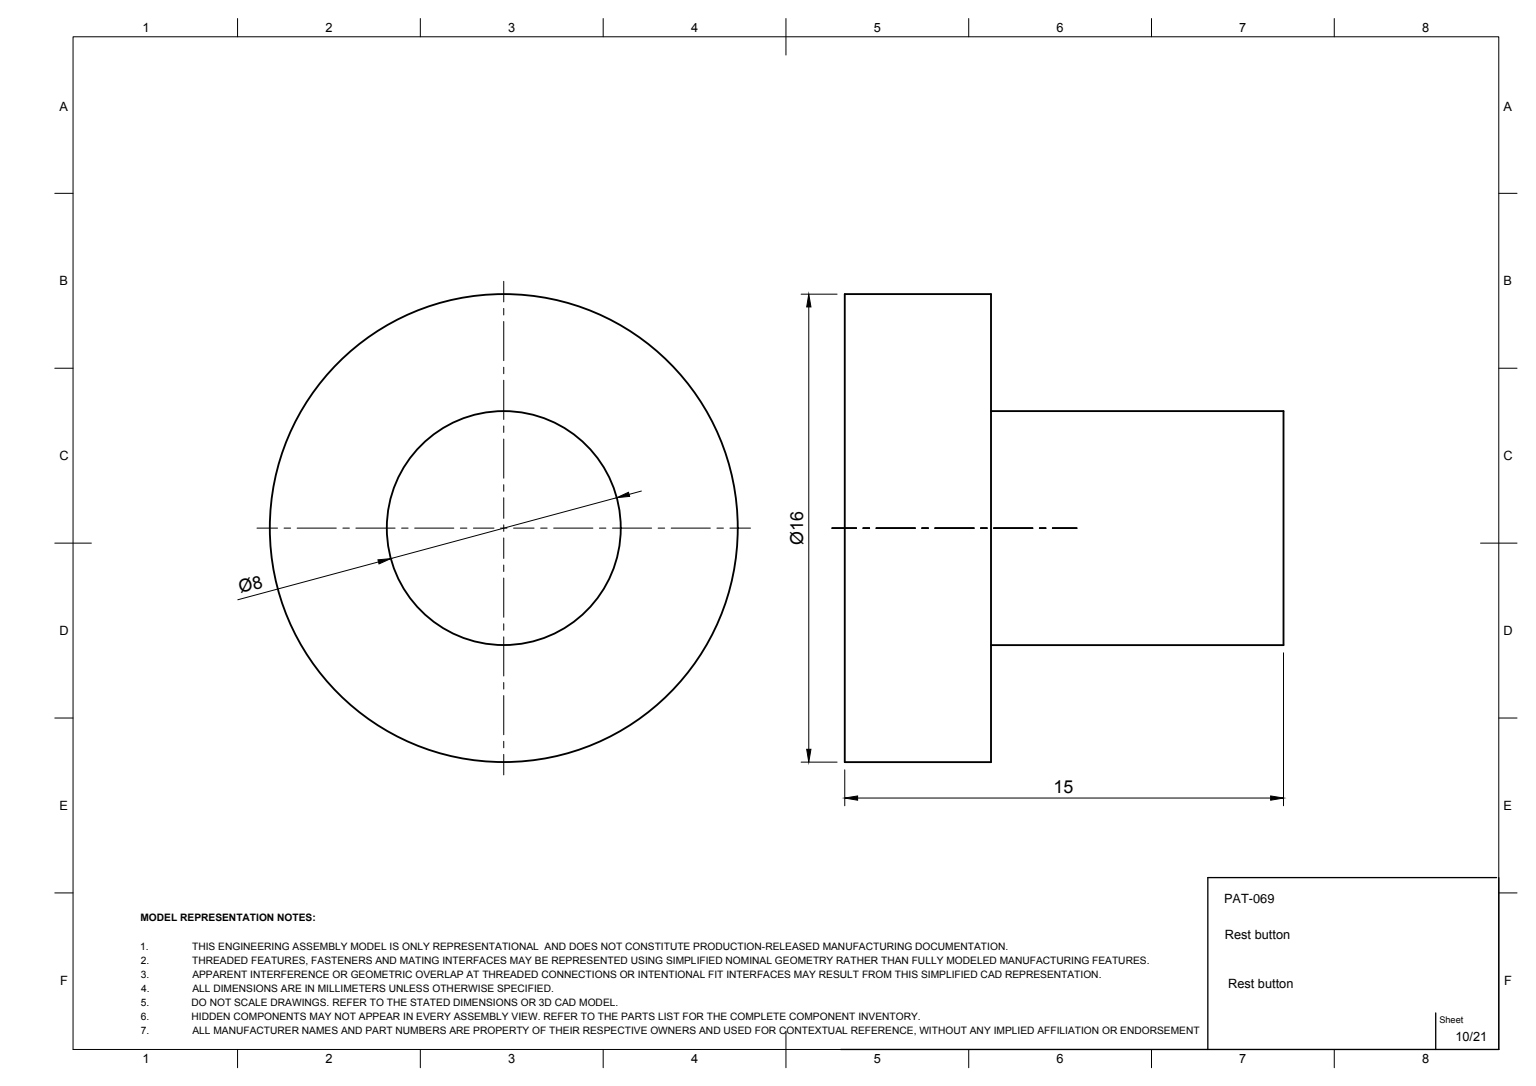
ISO-10303-21;
HEADER;
/* Generated by software containing ST-Developer
 * from STEP Tools, Inc. (www.steptools.com) 
 */

FILE_DESCRIPTION(
/* description */ ('Located fixture plate with toggle clamp'),
/* implementation_level */ '2;1');

FILE_NAME(
/* name */ 'Rest button.step',
/* time_stamp */ '2026-10-27T21:36:12-07:00',
/* author */ (''),
/* organization */ (''),
/* preprocessor_version */ 'ST-DEVELOPER v20.2',
/* originating_system */ 'Autodesk Translation Framework v15.17.0.0',
/* authorisation */ '');

FILE_SCHEMA (('AUTOMOTIVE_DESIGN { 1 0 10303 214 3 1 1 }'));
ENDSEC;

DATA;
#10=MECHANICAL_DESIGN_GEOMETRIC_PRESENTATION_REPRESENTATION('',(#329),#9285);
#281=SHAPE_REPRESENTATION_RELATIONSHIP('SRR','None',#9404,#305);
#305=ADVANCED_BREP_SHAPE_REPRESENTATION('',(#352),#9266);
#329=STYLED_ITEM('',(#9626),#352);
#352=MANIFOLD_SOLID_BREP('Body1',#5178);
#451=FACE_BOUND('',#1200,.T.);
#574=PLANE('',#5722);
#575=PLANE('',#5726);
#576=PLANE('',#5727);
#816=FACE_OUTER_BOUND('',#1196,.T.);
#817=FACE_OUTER_BOUND('',#1197,.T.);
#818=FACE_OUTER_BOUND('',#1198,.T.);
#819=FACE_OUTER_BOUND('',#1199,.T.);
#820=FACE_OUTER_BOUND('',#1201,.T.);
#1196=EDGE_LOOP('',(#4176,#4177,#4178,#4179));
#1197=EDGE_LOOP('',(#4180));
#1198=EDGE_LOOP('',(#4181,#4182,#4183,#4184));
#1199=EDGE_LOOP('',(#4185));
#1200=EDGE_LOOP('',(#4186));
#1201=EDGE_LOOP('',(#4187));
#1487=CIRCLE('',#5720,0.4);
#1488=CIRCLE('',#5721,0.4);
#1489=CIRCLE('',#5724,0.8);
#1490=CIRCLE('',#5725,0.8);
#1805=LINE('',#8343,#2215);
#1806=LINE('',#8350,#2216);
#2215=VECTOR('',#6773,0.4);
#2216=VECTOR('',#6782,0.8);
#2629=VERTEX_POINT('',#8340);
#2630=VERTEX_POINT('',#8342);
#2631=VERTEX_POINT('',#8347);
#2632=VERTEX_POINT('',#8349);
#3176=EDGE_CURVE('',#2629,#2629,#1487,.T.);
#3177=EDGE_CURVE('',#2629,#2630,#1805,.T.);
#3178=EDGE_CURVE('',#2630,#2630,#1488,.T.);
#3179=EDGE_CURVE('',#2631,#2631,#1489,.T.);
#3180=EDGE_CURVE('',#2631,#2632,#1806,.T.);
#3181=EDGE_CURVE('',#2632,#2632,#1490,.T.);
#4176=ORIENTED_EDGE('',*,*,#3176,.F.);
#4177=ORIENTED_EDGE('',*,*,#3177,.T.);
#4178=ORIENTED_EDGE('',*,*,#3178,.F.);
#4179=ORIENTED_EDGE('',*,*,#3177,.F.);
#4180=ORIENTED_EDGE('',*,*,#3176,.T.);
#4181=ORIENTED_EDGE('',*,*,#3179,.F.);
#4182=ORIENTED_EDGE('',*,*,#3180,.T.);
#4183=ORIENTED_EDGE('',*,*,#3181,.T.);
#4184=ORIENTED_EDGE('',*,*,#3180,.F.);
#4185=ORIENTED_EDGE('',*,*,#3179,.T.);
#4186=ORIENTED_EDGE('',*,*,#3178,.T.);
#4187=ORIENTED_EDGE('',*,*,#3181,.F.);
#4839=CYLINDRICAL_SURFACE('',#5719,0.4);
#4840=CYLINDRICAL_SURFACE('',#5723,0.8);
#5017=ADVANCED_FACE('',(#816),#4839,.T.);
#5018=ADVANCED_FACE('',(#817),#574,.T.);
#5019=ADVANCED_FACE('',(#818),#4840,.T.);
#5020=ADVANCED_FACE('',(#819,#451),#575,.T.);
#5021=ADVANCED_FACE('',(#820),#576,.F.);
#5178=CLOSED_SHELL('',(#5017,#5018,#5019,#5020,#5021));
#5718=AXIS2_PLACEMENT_3D('',#8338,#6767,#6768);
#5719=AXIS2_PLACEMENT_3D('',#8339,#6769,#6770);
#5720=AXIS2_PLACEMENT_3D('',#8341,#6771,#6772);
#5721=AXIS2_PLACEMENT_3D('',#8344,#6774,#6775);
#5722=AXIS2_PLACEMENT_3D('',#8345,#6776,#6777);
#5723=AXIS2_PLACEMENT_3D('',#8346,#6778,#6779);
#5724=AXIS2_PLACEMENT_3D('',#8348,#6780,#6781);
#5725=AXIS2_PLACEMENT_3D('',#8351,#6783,#6784);
#5726=AXIS2_PLACEMENT_3D('',#8352,#6785,#6786);
#5727=AXIS2_PLACEMENT_3D('',#8353,#6787,#6788);
#6767=DIRECTION('axis',(0.,0.,1.));
#6768=DIRECTION('refdir',(1.,0.,0.));
#6769=DIRECTION('center_axis',(1.,0.,0.));
#6770=DIRECTION('ref_axis',(0.,0.,-1.));
#6771=DIRECTION('center_axis',(1.,0.,0.));
#6772=DIRECTION('ref_axis',(0.,0.,-1.));
#6773=DIRECTION('',(-1.,0.,0.));
#6774=DIRECTION('center_axis',(-1.,0.,0.));
#6775=DIRECTION('ref_axis',(0.,0.,-1.));
#6776=DIRECTION('center_axis',(1.,0.,0.));
#6777=DIRECTION('ref_axis',(0.,0.,-1.));
#6778=DIRECTION('center_axis',(1.,0.,0.));
#6779=DIRECTION('ref_axis',(0.,0.,-1.));
#6780=DIRECTION('center_axis',(1.,0.,0.));
#6781=DIRECTION('ref_axis',(0.,0.,-1.));
#6782=DIRECTION('',(-1.,0.,0.));
#6783=DIRECTION('center_axis',(1.,0.,0.));
#6784=DIRECTION('ref_axis',(0.,0.,-1.));
#6785=DIRECTION('center_axis',(1.,0.,0.));
#6786=DIRECTION('ref_axis',(0.,0.,-1.));
#6787=DIRECTION('center_axis',(1.,0.,0.));
#6788=DIRECTION('ref_axis',(0.,0.,-1.));
#8338=CARTESIAN_POINT('',(0.,0.,0.));
#8339=CARTESIAN_POINT('Origin',(18.8,-2.5,2.));
#8340=CARTESIAN_POINT('',(19.8,-2.5,2.4));
#8341=CARTESIAN_POINT('Origin',(19.8,-2.5,2.));
#8342=CARTESIAN_POINT('',(18.8,-2.5,2.4));
#8343=CARTESIAN_POINT('',(18.8,-2.5,2.4));
#8344=CARTESIAN_POINT('Origin',(18.8,-2.5,2.));
#8345=CARTESIAN_POINT('Origin',(19.8,-2.5,2.));
#8346=CARTESIAN_POINT('Origin',(18.3,-2.5,2.));
#8347=CARTESIAN_POINT('',(18.8,-2.5,2.8));
#8348=CARTESIAN_POINT('Origin',(18.8,-2.5,2.));
#8349=CARTESIAN_POINT('',(18.3,-2.5,2.8));
#8350=CARTESIAN_POINT('',(18.3,-2.5,2.8));
#8351=CARTESIAN_POINT('Origin',(18.3,-2.5,2.));
#8352=CARTESIAN_POINT('Origin',(18.8,-2.5,2.));
#8353=CARTESIAN_POINT('Origin',(18.3,-2.5,2.));
#9236=UNCERTAINTY_MEASURE_WITH_UNIT(LENGTH_MEASURE(0.001),#9286,
'DISTANCE_ACCURACY_VALUE',
'Maximum model space distance between geometric entities at asserted c
onnectivities');
#9255=UNCERTAINTY_MEASURE_WITH_UNIT(LENGTH_MEASURE(0.001),#9286,
'DISTANCE_ACCURACY_VALUE',
'Maximum model space distance between geometric entities at asserted c
onnectivities');
#9266=(
GEOMETRIC_REPRESENTATION_CONTEXT(3)
GLOBAL_UNCERTAINTY_ASSIGNED_CONTEXT((#9236))
GLOBAL_UNIT_ASSIGNED_CONTEXT((#9286,#9288,#9289))
REPRESENTATION_CONTEXT('','3D')
);
#9285=(
GEOMETRIC_REPRESENTATION_CONTEXT(3)
GLOBAL_UNCERTAINTY_ASSIGNED_CONTEXT((#9255))
GLOBAL_UNIT_ASSIGNED_CONTEXT((#9286,#9288,#9289))
REPRESENTATION_CONTEXT('','3D')
);
#9286=(
LENGTH_UNIT()
NAMED_UNIT(*)
SI_UNIT(.CENTI.,.METRE.)
);
#9288=(
NAMED_UNIT(*)
PLANE_ANGLE_UNIT()
SI_UNIT($,.RADIAN.)
);
#9289=(
NAMED_UNIT(*)
SI_UNIT($,.STERADIAN.)
SOLID_ANGLE_UNIT()
);
#9300=SHAPE_DEFINITION_REPRESENTATION(#9329,#9404);
#9329=PRODUCT_DEFINITION_SHAPE('',$,#9434);
#9404=SHAPE_REPRESENTATION('',(#5718),#9266);
#9423=PRODUCT_DEFINITION_CONTEXT('part definition',#9512,'design');
#9434=PRODUCT_DEFINITION('Rest button','Rest button',#9463,#9423);
#9463=PRODUCT_DEFINITION_FORMATION('',$,#9524);
#9512=APPLICATION_CONTEXT(
'Core Data for Automotive Mechanical Design Process');
#9513=PRODUCT_CONTEXT('part definition',#9512,'mechanical');
#9524=PRODUCT('Rest button','Rest button','Rest button',(#9513));
#9620=COLOUR_RGB('Off White',0.89,0.88,0.83);
#9621=FILL_AREA_STYLE_COLOUR('',#9620);
#9622=FILL_AREA_STYLE('',(#9621));
#9623=SURFACE_STYLE_FILL_AREA(#9622);
#9624=SURFACE_SIDE_STYLE('',(#9623));
#9625=SURFACE_STYLE_USAGE(.BOTH.,#9624);
#9626=PRESENTATION_STYLE_ASSIGNMENT((#9625));
ENDSEC;
END-ISO-10303-21;
